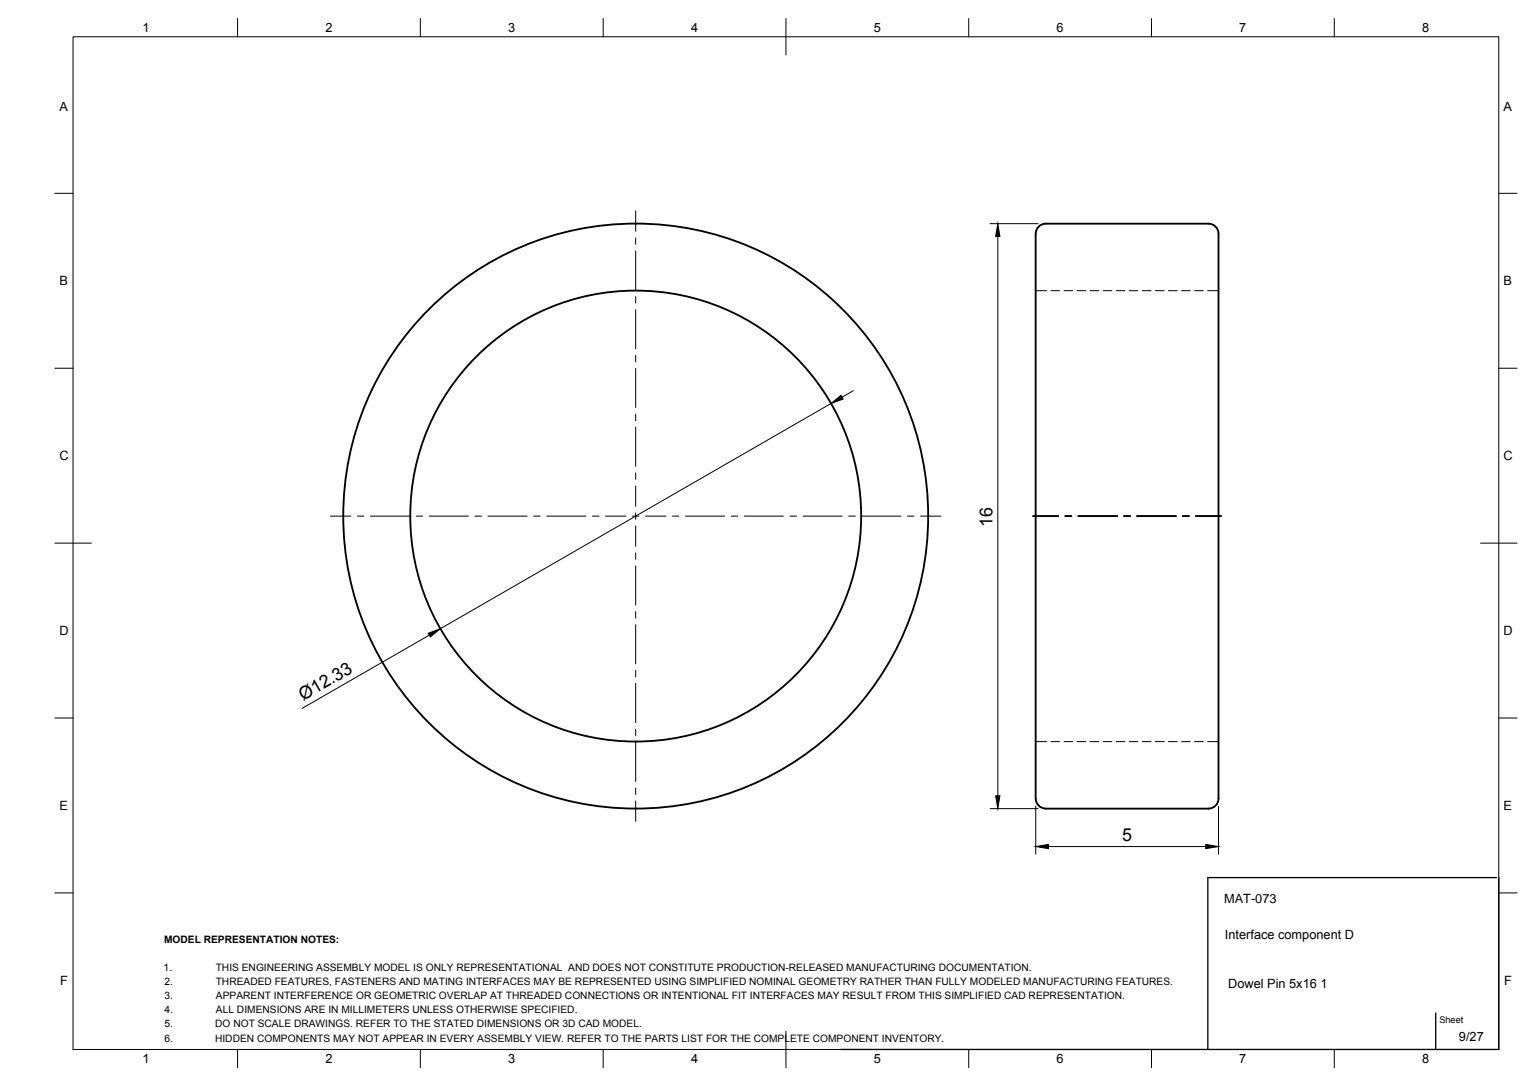
ISO-10303-21;
HEADER;
/* Generated by software containing ST-Developer
 * from STEP Tools, Inc. (www.steptools.com) 
 */

FILE_DESCRIPTION(
/* description */ ('CAx-IF Rec.Pracs.---Representation and Presentation of Product Manufa
cturing Information (PMI)---4.0---2014-10-13'),
/* implementation_level */ '2;1');

FILE_NAME(
/* name */ 'Interface component D.step',
/* time_stamp */ '2026-10-24T18:52:33-07:00',
/* author */ (''),
/* organization */ (''),
/* preprocessor_version */ 'ST-DEVELOPER v20.2',
/* originating_system */ 'Autodesk Translation Framework v15.17.0.0',
/* authorisation */ '');

FILE_SCHEMA (('AP242_MANAGED_MODEL_BASED_3D_ENGINEERING_MIM_LF { 1 0 10303 442 2 1 4 }'));
ENDSEC;

DATA;
#10=MECHANICAL_DESIGN_GEOMETRIC_PRESENTATION_REPRESENTATION('',(#420),#34876);
#354=SHAPE_REPRESENTATION_RELATIONSHIP('SRR','None',#34991,#387);
#387=ADVANCED_BREP_SHAPE_REPRESENTATION('',(#453),#34849);
#420=STYLED_ITEM('',(#35161),#453);
#453=MANIFOLD_SOLID_BREP('Dowel Pin 5x16 1',#19560);
#517=FACE_BOUND('',#6255,.T.);
#518=FACE_BOUND('',#6258,.T.);
#776=PLANE('',#20801);
#777=PLANE('',#20806);
#1637=LINE('',#30872,#3236);
#1638=LINE('',#30887,#3237);
#3236=VECTOR('',#24508,0.008);
#3237=VECTOR('',#24529,0.00616666666666666);
#4464=CYLINDRICAL_SURFACE('',#20798,0.008);
#4465=CYLINDRICAL_SURFACE('',#20808,0.00616666666666666);
#5170=FACE_OUTER_BOUND('',#6252,.T.);
#5171=FACE_OUTER_BOUND('',#6253,.T.);
#5172=FACE_OUTER_BOUND('',#6254,.T.);
#5173=FACE_OUTER_BOUND('',#6256,.T.);
#5174=FACE_OUTER_BOUND('',#6257,.T.);
#5175=FACE_OUTER_BOUND('',#6259,.T.);
#6252=EDGE_LOOP('',(#14868,#14869,#14870,#14871,#14872));
#6253=EDGE_LOOP('',(#14873,#14874,#14875,#14876,#14877,#14878));
#6254=EDGE_LOOP('',(#14879));
#6255=EDGE_LOOP('',(#14880));
#6256=EDGE_LOOP('',(#14881,#14882,#14883,#14884,#14885));
#6257=EDGE_LOOP('',(#14886));
#6258=EDGE_LOOP('',(#14887));
#6259=EDGE_LOOP('',(#14888,#14889,#14890,#14891));
#7362=CIRCLE('',#20794,0.00772500000001);
#7363=CIRCLE('',#20795,0.000275);
#7364=CIRCLE('',#20796,0.00800000000001);
#7365=CIRCLE('',#20797,0.00800000000001);
#7366=CIRCLE('',#20799,0.00800000000001);
#7367=CIRCLE('',#20800,0.00800000000001);
#7368=CIRCLE('',#20802,0.00616666666667666);
#7369=CIRCLE('',#20804,0.000275);
#7370=CIRCLE('',#20805,0.00772500000001);
#7371=CIRCLE('',#20807,0.00616666666667666);
#8756=VERTEX_POINT('',#30863);
#8757=VERTEX_POINT('',#30865);
#8758=VERTEX_POINT('',#30867);
#8759=VERTEX_POINT('',#30871);
#8760=VERTEX_POINT('',#30873);
#8761=VERTEX_POINT('',#30877);
#8762=VERTEX_POINT('',#30880);
#8763=VERTEX_POINT('',#30884);
#10992=EDGE_CURVE('',#8756,#8756,#7362,.T.);
#10993=EDGE_CURVE('',#8756,#8757,#7363,.T.);
#10994=EDGE_CURVE('',#8757,#8758,#7364,.T.);
#10995=EDGE_CURVE('',#8758,#8757,#7365,.T.);
#10996=EDGE_CURVE('',#8758,#8759,#1637,.T.);
#10997=EDGE_CURVE('',#8760,#8759,#7366,.T.);
#10998=EDGE_CURVE('',#8759,#8760,#7367,.T.);
#10999=EDGE_CURVE('',#8761,#8761,#7368,.T.);
#11000=EDGE_CURVE('',#8760,#8762,#7369,.T.);
#11001=EDGE_CURVE('',#8762,#8762,#7370,.T.);
#11002=EDGE_CURVE('',#8763,#8763,#7371,.T.);
#11003=EDGE_CURVE('',#8763,#8761,#1638,.T.);
#14868=ORIENTED_EDGE('',*,*,#10992,.T.);
#14869=ORIENTED_EDGE('',*,*,#10993,.T.);
#14870=ORIENTED_EDGE('',*,*,#10994,.T.);
#14871=ORIENTED_EDGE('',*,*,#10995,.T.);
#14872=ORIENTED_EDGE('',*,*,#10993,.F.);
#14873=ORIENTED_EDGE('',*,*,#10995,.F.);
#14874=ORIENTED_EDGE('',*,*,#10996,.T.);
#14875=ORIENTED_EDGE('',*,*,#10997,.F.);
#14876=ORIENTED_EDGE('',*,*,#10998,.F.);
#14877=ORIENTED_EDGE('',*,*,#10996,.F.);
#14878=ORIENTED_EDGE('',*,*,#10994,.F.);
#14879=ORIENTED_EDGE('',*,*,#10992,.F.);
#14880=ORIENTED_EDGE('',*,*,#10999,.F.);
#14881=ORIENTED_EDGE('',*,*,#10998,.T.);
#14882=ORIENTED_EDGE('',*,*,#11000,.T.);
#14883=ORIENTED_EDGE('',*,*,#11001,.T.);
#14884=ORIENTED_EDGE('',*,*,#11000,.F.);
#14885=ORIENTED_EDGE('',*,*,#10997,.T.);
#14886=ORIENTED_EDGE('',*,*,#11001,.F.);
#14887=ORIENTED_EDGE('',*,*,#11002,.T.);
#14888=ORIENTED_EDGE('',*,*,#11002,.F.);
#14889=ORIENTED_EDGE('',*,*,#11003,.T.);
#14890=ORIENTED_EDGE('',*,*,#10999,.T.);
#14891=ORIENTED_EDGE('',*,*,#11003,.F.);
#18498=TOROIDAL_SURFACE('',#20793,0.007725,0.000275);
#18499=TOROIDAL_SURFACE('',#20803,0.007725,0.000275);
#18886=ADVANCED_FACE('',(#5170),#18498,.T.);
#18887=ADVANCED_FACE('',(#5171),#4464,.T.);
#18888=ADVANCED_FACE('',(#5172,#517),#776,.T.);
#18889=ADVANCED_FACE('',(#5173),#18499,.T.);
#18890=ADVANCED_FACE('',(#5174,#518),#777,.T.);
#18891=ADVANCED_FACE('',(#5175),#4465,.F.);
#19560=CLOSED_SHELL('',(#18886,#18887,#18888,#18889,#18890,#18891));
#20792=AXIS2_PLACEMENT_3D('',#30861,#24494,#24495);
#20793=AXIS2_PLACEMENT_3D('',#30862,#24496,#24497);
#20794=AXIS2_PLACEMENT_3D('',#30864,#24498,#24499);
#20795=AXIS2_PLACEMENT_3D('',#30866,#24500,#24501);
#20796=AXIS2_PLACEMENT_3D('',#30868,#24502,#24503);
#20797=AXIS2_PLACEMENT_3D('',#30869,#24504,#24505);
#20798=AXIS2_PLACEMENT_3D('',#30870,#24506,#24507);
#20799=AXIS2_PLACEMENT_3D('',#30874,#24509,#24510);
#20800=AXIS2_PLACEMENT_3D('',#30875,#24511,#24512);
#20801=AXIS2_PLACEMENT_3D('',#30876,#24513,#24514);
#20802=AXIS2_PLACEMENT_3D('',#30878,#24515,#24516);
#20803=AXIS2_PLACEMENT_3D('',#30879,#24517,#24518);
#20804=AXIS2_PLACEMENT_3D('',#30881,#24519,#24520);
#20805=AXIS2_PLACEMENT_3D('',#30882,#24521,#24522);
#20806=AXIS2_PLACEMENT_3D('',#30883,#24523,#24524);
#20807=AXIS2_PLACEMENT_3D('',#30885,#24525,#24526);
#20808=AXIS2_PLACEMENT_3D('',#30886,#24527,#24528);
#24494=DIRECTION('axis',(0.,0.,1.));
#24495=DIRECTION('refdir',(1.,0.,0.));
#24496=DIRECTION('center_axis',(6.12323404134149E-17,-1.,3.14444500472474E-32));
#24497=DIRECTION('ref_axis',(1.55749764652046E-5,0.,-0.99999999987871));
#24498=DIRECTION('center_axis',(-6.12323404134149E-17,1.,-3.14444500472474E-32));
#24499=DIRECTION('ref_axis',(-0.99999999987871,-6.1232340405988E-17,-1.55749751705838E-5));
#24500=DIRECTION('center_axis',(-0.99999999987871,-6.12323404059881E-17,
-1.55749764653271E-5));
#24501=DIRECTION('ref_axis',(-1.55749764653271E-5,0.,0.99999999987871));
#24502=DIRECTION('center_axis',(6.12323404134149E-17,-1.,3.14444500472474E-32));
#24503=DIRECTION('ref_axis',(-0.99999999987871,-6.12323404059881E-17,-1.55749752150822E-5));
#24504=DIRECTION('center_axis',(6.12323404134149E-17,-1.,3.14444500472474E-32));
#24505=DIRECTION('ref_axis',(-0.99999999987871,-6.12323404059881E-17,-1.55749752150822E-5));
#24506=DIRECTION('center_axis',(6.12323404134149E-17,-1.,3.14444500472474E-32));
#24507=DIRECTION('ref_axis',(0.99999999987871,6.12323404059881E-17,1.55749764652046E-5));
#24508=DIRECTION('',(-6.12323404134149E-17,1.,-3.14444500472474E-32));
#24509=DIRECTION('center_axis',(-6.12323404134149E-17,1.,-3.14444500472474E-32));
#24510=DIRECTION('ref_axis',(-0.99999999987871,-6.12323404059881E-17,-1.55749752150822E-5));
#24511=DIRECTION('center_axis',(-6.12323404134149E-17,1.,-3.14444500472474E-32));
#24512=DIRECTION('ref_axis',(-0.99999999987871,-6.12323404059881E-17,-1.55749752150822E-5));
#24513=DIRECTION('center_axis',(6.12323404134149E-17,-1.,3.14444500472474E-32));
#24514=DIRECTION('ref_axis',(0.99999999987871,6.12323404059881E-17,1.55749764652046E-5));
#24515=DIRECTION('center_axis',(6.12323404134149E-17,-1.,3.14444500472474E-32));
#24516=DIRECTION('ref_axis',(0.99999999987871,6.1232340405988E-17,1.55749764652046E-5));
#24517=DIRECTION('center_axis',(6.12323404134149E-17,-1.,3.14444500472474E-32));
#24518=DIRECTION('ref_axis',(1.55749764652046E-5,0.,-0.99999999987871));
#24519=DIRECTION('center_axis',(-0.99999999987871,-6.12323404059881E-17,
-1.55749764653271E-5));
#24520=DIRECTION('ref_axis',(-1.55749764653271E-5,0.,0.99999999987871));
#24521=DIRECTION('center_axis',(6.12323404134149E-17,-1.,3.14444500472474E-32));
#24522=DIRECTION('ref_axis',(-0.99999999987871,-6.1232340405988E-17,-1.55749751705838E-5));
#24523=DIRECTION('center_axis',(-6.12323404134149E-17,1.,-3.14444500472474E-32));
#24524=DIRECTION('ref_axis',(-1.55749764652046E-5,-9.53692260816889E-22,
0.99999999987871));
#24525=DIRECTION('center_axis',(6.12323404134149E-17,-1.,3.14444500472474E-32));
#24526=DIRECTION('ref_axis',(0.99999999987871,6.1232340405988E-17,1.55749764652046E-5));
#24527=DIRECTION('center_axis',(6.12323404134149E-17,-1.,3.14444500472474E-32));
#24528=DIRECTION('ref_axis',(0.99999999987871,6.1232340405988E-17,1.55749764652046E-5));
#24529=DIRECTION('',(6.12323404134149E-17,-1.,3.14444500472474E-32));
#30861=CARTESIAN_POINT('',(0.,0.,0.));
#30862=CARTESIAN_POINT('Origin',(-4.34919666873154E-17,-0.030975,7.19534755436855E-33));
#30863=CARTESIAN_POINT('',(-1.20316693238282E-7,-0.03125000000001,0.00772499999907304));
#30864=CARTESIAN_POINT('Origin',(-4.34751277937011E-17,-0.03125000000001,
7.20399477813186E-33));
#30865=CARTESIAN_POINT('',(-1.24599811766264E-7,-0.03097500000001,0.00799999999903968));
#30866=CARTESIAN_POINT('Origin',(-1.20316693238144E-7,-0.030975,0.00772499999906304));
#30867=CARTESIAN_POINT('',(-0.00799999999903972,-0.03097500000001,-1.24599801720813E-7));
#30868=CARTESIAN_POINT('Origin',(-4.34919666873148E-17,-0.03097500000001,
7.19534755436887E-33));
#30869=CARTESIAN_POINT('Origin',(-4.34919666873148E-17,-0.03097500000001,
7.19534755436887E-33));
#30870=CARTESIAN_POINT('Origin',(-4.36282086447352E-17,-0.02875,7.12538365301343E-33));
#30871=CARTESIAN_POINT('',(-0.00799999999903972,-0.02652500000001,-1.24599801720813E-7));
#30872=CARTESIAN_POINT('',(-0.00799999999902972,-0.02875,-1.24599811722617E-7));
#30873=CARTESIAN_POINT('',(-1.24599811766537E-7,-0.02652500000001,0.00799999999903968));
#30874=CARTESIAN_POINT('Origin',(-4.37644506021545E-17,-0.02652500000001,
7.05541975165862E-33));
#30875=CARTESIAN_POINT('Origin',(-4.37644506021545E-17,-0.02652500000001,
7.05541975165862E-33));
#30876=CARTESIAN_POINT('Origin',(0.00708333333247415,-0.03125,1.10322749961866E-7));
#30877=CARTESIAN_POINT('',(-0.00616666666591875,-0.03125000000001,-9.60456882028501E-8));
#30878=CARTESIAN_POINT('Origin',(-4.34751277937011E-17,-0.03125000000001,
7.20399477813186E-33));
#30879=CARTESIAN_POINT('Origin',(-4.37644506021551E-17,-0.026525,7.0554197516583E-33));
#30880=CARTESIAN_POINT('',(-1.20316693238589E-7,-0.02625000000001,0.00772499999907304));
#30881=CARTESIAN_POINT('Origin',(-1.20316693238416E-7,-0.026525,0.00772499999906304));
#30882=CARTESIAN_POINT('Origin',(-4.37812894957682E-17,-0.02625000000001,
7.04677252789562E-33));
#30883=CARTESIAN_POINT('Origin',(0.00708333333247415,-0.02625,1.10322749961866E-7));
#30884=CARTESIAN_POINT('',(-0.00616666666591875,-0.02625000000001,-9.60456882028501E-8));
#30885=CARTESIAN_POINT('Origin',(-4.37812894957682E-17,-0.02625000000001,
7.04677252789562E-33));
#30886=CARTESIAN_POINT('Origin',(-4.36282086447352E-17,-0.02875,7.12538365301343E-33));
#30887=CARTESIAN_POINT('',(-0.00616666666591875,-0.02875,-9.60456882028501E-8));
#34814=UNCERTAINTY_MEASURE_WITH_UNIT(LENGTH_MEASURE(1.E-5),#34877,
'DISTANCE_ACCURACY_VALUE',
'Maximum model space distance between geometric entities at asserted c
onnectivities');
#34841=UNCERTAINTY_MEASURE_WITH_UNIT(LENGTH_MEASURE(1.E-5),#34877,
'DISTANCE_ACCURACY_VALUE',
'Maximum model space distance between geometric entities at asserted c
onnectivities');
#34849=(
GEOMETRIC_REPRESENTATION_CONTEXT(3)
GLOBAL_UNCERTAINTY_ASSIGNED_CONTEXT((#34814))
GLOBAL_UNIT_ASSIGNED_CONTEXT((#34877,#34878,#34879))
REPRESENTATION_CONTEXT('','3D')
);
#34876=(
GEOMETRIC_REPRESENTATION_CONTEXT(3)
GLOBAL_UNCERTAINTY_ASSIGNED_CONTEXT((#34841))
GLOBAL_UNIT_ASSIGNED_CONTEXT((#34877,#34878,#34879))
REPRESENTATION_CONTEXT('','3D')
);
#34877=(
LENGTH_UNIT()
NAMED_UNIT(*)
SI_UNIT($,.METRE.)
);
#34878=(
NAMED_UNIT(*)
PLANE_ANGLE_UNIT()
SI_UNIT($,.RADIAN.)
);
#34879=(
NAMED_UNIT(*)
SI_UNIT($,.STERADIAN.)
SOLID_ANGLE_UNIT()
);
#34887=SHAPE_DEFINITION_REPRESENTATION(#34921,#34991);
#34921=PRODUCT_DEFINITION_SHAPE('',$,#35026);
#34991=SHAPE_REPRESENTATION('',(#20792),#34849);
#35018=PRODUCT_DEFINITION_CONTEXT('part definition',#35122,'design');
#35026=PRODUCT_DEFINITION('Interface component D',
'Interface component D',#35060,#35018);
#35060=PRODUCT_DEFINITION_FORMATION('',$,#35131);
#35122=APPLICATION_CONTEXT('Managed model based 3d engineering');
#35123=PRODUCT_CONTEXT('part definition',#35122,'mechanical');
#35131=PRODUCT('Interface component D','Interface component D',
'LEGAL AND USAGE DISCLAIMER: this Data/Model is provided \X2\201C\X0\A
S IS\X2\201D\X0\ for informational and representational only. It is a 
geometric approximation and is NOT engineered, certified, or guarantee
d for dimensional accuracy, exact tolerances, or production-level prec
ision. Vendor disclaims all implied warranties including fitness for a
 particular purpose. DO NOT USE FOR DIRECT PHYSICAL MANUFACTURING, AUT
OMATED PRODUCTION, OR SAFETY-CRITICAL SYSTEMS without independent engi
neering verification and resolution of any design discrepancies.',(#35123));
#35161=PRESENTATION_STYLE_ASSIGNMENT((#35170));
#35170=SURFACE_STYLE_USAGE(.BOTH.,#35179);
#35179=SURFACE_SIDE_STYLE('',(#35188));
#35188=SURFACE_STYLE_FILL_AREA(#35197);
#35197=FILL_AREA_STYLE('Aluminum - Anodized Glossy (Blue)',(#35206));
#35206=FILL_AREA_STYLE_COLOUR('Aluminum - Anodized Glossy (Blue)',#35215);
#35215=COLOUR_RGB('Aluminum - Anodized Glossy (Blue)',0.349019607843137,
0.584313725490196,0.854901960784314);
ENDSEC;
END-ISO-10303-21;
